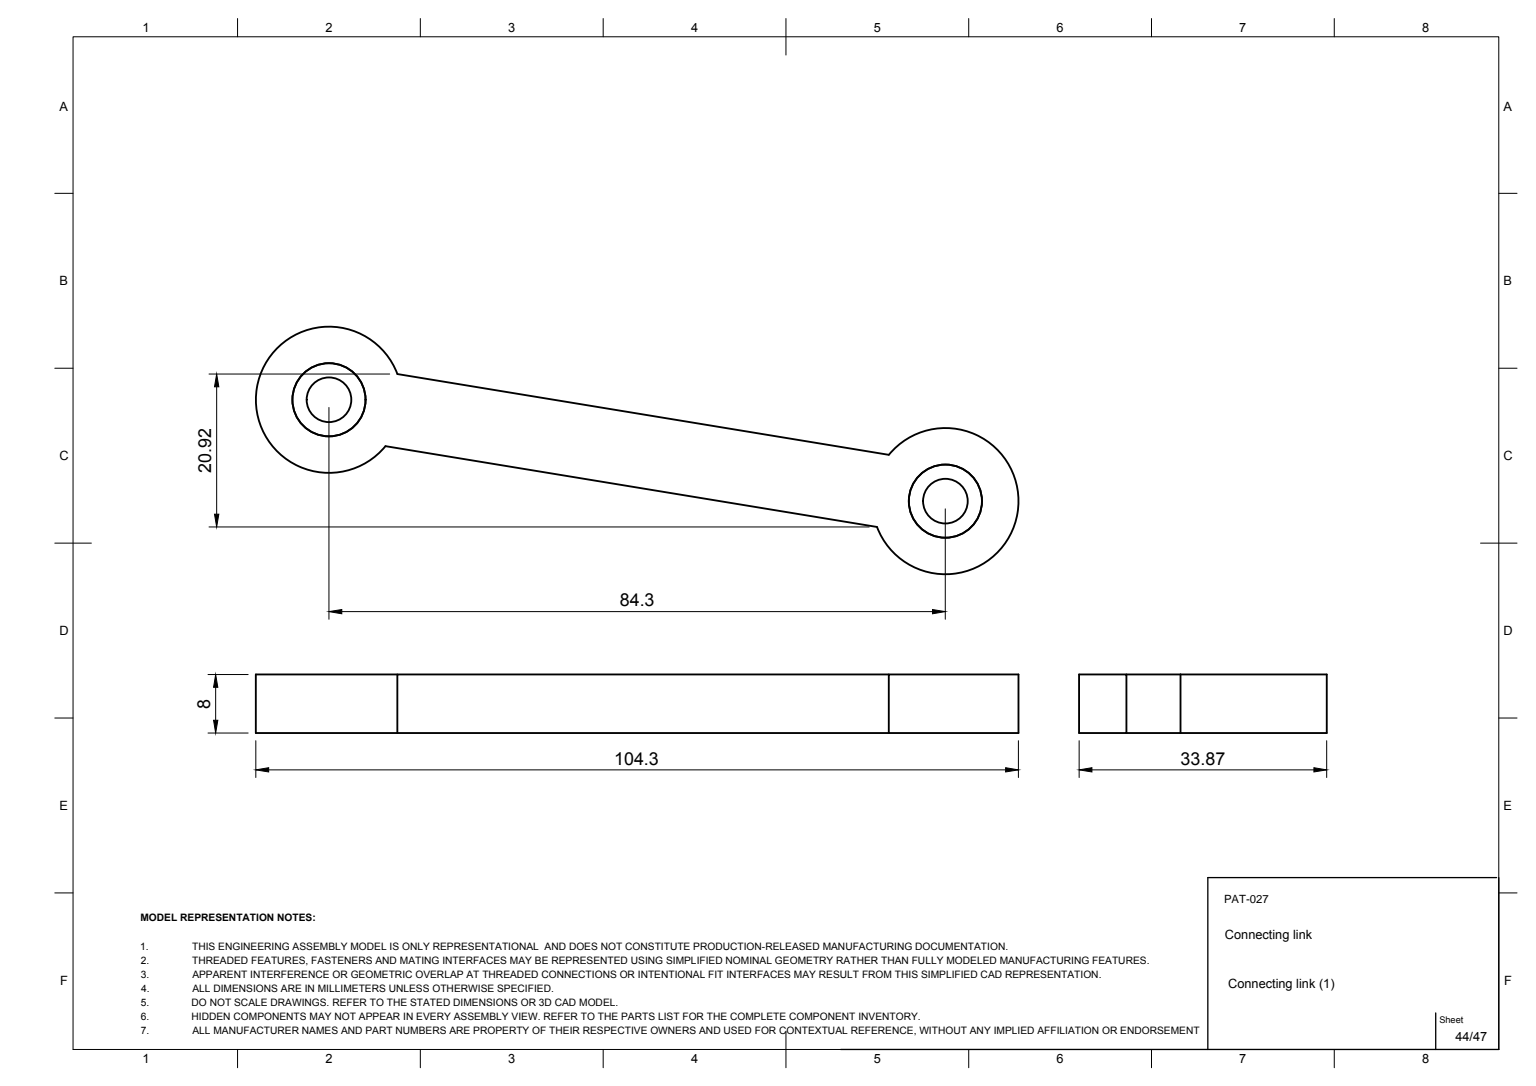
ISO-10303-21;
HEADER;
/* Generated by software containing ST-Developer
 * from STEP Tools, Inc. (www.steptools.com) 
 */

FILE_DESCRIPTION(
/* description */ ('Crank-driven oscillating fan base (mechanism only)'),

/* implementation_level */ '2;1');

FILE_NAME(
/* name */ 'Connecting link.step',
/* time_stamp */ '2026-10-28T03:25:00-07:00',
/* author */ (''),
/* organization */ (''),
/* preprocessor_version */ 'ST-DEVELOPER v20.2',
/* originating_system */ 'Autodesk Translation Framework v15.17.0.0',
/* authorisation */ '');

FILE_SCHEMA (('AUTOMOTIVE_DESIGN { 1 0 10303 214 3 1 1 }'));
ENDSEC;

DATA;
#10=MECHANICAL_DESIGN_GEOMETRIC_PRESENTATION_REPRESENTATION('',(#482),#11916);
#394=SHAPE_REPRESENTATION_RELATIONSHIP('SRR','None',#12122,#434);
#434=ADVANCED_BREP_SHAPE_REPRESENTATION('',(#527),#11913);
#482=STYLED_ITEM('',(#12368),#527);
#527=MANIFOLD_SOLID_BREP('Body1',#6115);
#684=FACE_BOUND('',#1779,.T.);
#685=FACE_BOUND('',#1780,.T.);
#686=FACE_BOUND('',#1784,.T.);
#687=FACE_BOUND('',#1785,.T.);
#878=PLANE('',#7379);
#879=PLANE('',#7380);
#880=PLANE('',#7382);
#881=PLANE('',#7385);
#1245=FACE_OUTER_BOUND('',#1774,.T.);
#1246=FACE_OUTER_BOUND('',#1775,.T.);
#1247=FACE_OUTER_BOUND('',#1776,.T.);
#1248=FACE_OUTER_BOUND('',#1777,.T.);
#1249=FACE_OUTER_BOUND('',#1778,.T.);
#1250=FACE_OUTER_BOUND('',#1781,.T.);
#1251=FACE_OUTER_BOUND('',#1782,.T.);
#1252=FACE_OUTER_BOUND('',#1783,.T.);
#1774=EDGE_LOOP('',(#5486,#5487,#5488,#5489));
#1775=EDGE_LOOP('',(#5490,#5491,#5492,#5493));
#1776=EDGE_LOOP('',(#5494,#5495,#5496,#5497));
#1777=EDGE_LOOP('',(#5498,#5499,#5500,#5501));
#1778=EDGE_LOOP('',(#5502,#5503,#5504,#5505));
#1779=EDGE_LOOP('',(#5506));
#1780=EDGE_LOOP('',(#5507));
#1781=EDGE_LOOP('',(#5508,#5509,#5510,#5511));
#1782=EDGE_LOOP('',(#5512,#5513,#5514,#5515));
#1783=EDGE_LOOP('',(#5516,#5517,#5518,#5519));
#1784=EDGE_LOOP('',(#5520));
#1785=EDGE_LOOP('',(#5521));
#2117=LINE('',#11752,#2450);
#2118=LINE('',#11758,#2451);
#2119=LINE('',#11763,#2452);
#2120=LINE('',#11767,#2453);
#2121=LINE('',#11771,#2454);
#2122=LINE('',#11773,#2455);
#2123=LINE('',#11774,#2456);
#2124=LINE('',#11777,#2457);
#2125=LINE('',#11781,#2458);
#2126=LINE('',#11782,#2459);
#2450=VECTOR('',#9356,0.5);
#2451=VECTOR('',#9363,0.5);
#2452=VECTOR('',#9368,1.);
#2453=VECTOR('',#9371,1.);
#2454=VECTOR('',#9376,1.);
#2455=VECTOR('',#9377,1.);
#2456=VECTOR('',#9378,1.);
#2457=VECTOR('',#9381,1.);
#2458=VECTOR('',#9386,1.);
#2459=VECTOR('',#9387,1.);
#2813=CIRCLE('',#7371,0.5);
#2814=CIRCLE('',#7372,0.5);
#2815=CIRCLE('',#7374,0.5);
#2816=CIRCLE('',#7375,0.5);
#2817=CIRCLE('',#7377,1.);
#2818=CIRCLE('',#7378,1.);
#2819=CIRCLE('',#7381,1.);
#2820=CIRCLE('',#7384,1.);
#3309=VERTEX_POINT('',#11749);
#3310=VERTEX_POINT('',#11751);
#3311=VERTEX_POINT('',#11755);
#3312=VERTEX_POINT('',#11757);
#3313=VERTEX_POINT('',#11761);
#3314=VERTEX_POINT('',#11762);
#3315=VERTEX_POINT('',#11764);
#3316=VERTEX_POINT('',#11766);
#3317=VERTEX_POINT('',#11770);
#3318=VERTEX_POINT('',#11772);
#3319=VERTEX_POINT('',#11776);
#3320=VERTEX_POINT('',#11780);
#4038=EDGE_CURVE('',#3309,#3309,#2813,.T.);
#4039=EDGE_CURVE('',#3309,#3310,#2117,.T.);
#4040=EDGE_CURVE('',#3310,#3310,#2814,.T.);
#4041=EDGE_CURVE('',#3311,#3311,#2815,.T.);
#4042=EDGE_CURVE('',#3311,#3312,#2118,.T.);
#4043=EDGE_CURVE('',#3312,#3312,#2816,.T.);
#4044=EDGE_CURVE('',#3313,#3314,#2119,.T.);
#4045=EDGE_CURVE('',#3315,#3313,#2817,.T.);
#4046=EDGE_CURVE('',#3316,#3315,#2120,.T.);
#4047=EDGE_CURVE('',#3316,#3314,#2818,.T.);
#4048=EDGE_CURVE('',#3317,#3314,#2121,.T.);
#4049=EDGE_CURVE('',#3318,#3317,#2122,.T.);
#4050=EDGE_CURVE('',#3313,#3318,#2123,.T.);
#4051=EDGE_CURVE('',#3316,#3319,#2124,.T.);
#4052=EDGE_CURVE('',#3317,#3319,#2819,.T.);
#4053=EDGE_CURVE('',#3320,#3315,#2125,.T.);
#4054=EDGE_CURVE('',#3319,#3320,#2126,.T.);
#4055=EDGE_CURVE('',#3318,#3320,#2820,.T.);
#5486=ORIENTED_EDGE('',*,*,#4038,.F.);
#5487=ORIENTED_EDGE('',*,*,#4039,.T.);
#5488=ORIENTED_EDGE('',*,*,#4040,.F.);
#5489=ORIENTED_EDGE('',*,*,#4039,.F.);
#5490=ORIENTED_EDGE('',*,*,#4041,.F.);
#5491=ORIENTED_EDGE('',*,*,#4042,.T.);
#5492=ORIENTED_EDGE('',*,*,#4043,.F.);
#5493=ORIENTED_EDGE('',*,*,#4042,.F.);
#5494=ORIENTED_EDGE('',*,*,#4044,.F.);
#5495=ORIENTED_EDGE('',*,*,#4045,.F.);
#5496=ORIENTED_EDGE('',*,*,#4046,.F.);
#5497=ORIENTED_EDGE('',*,*,#4047,.T.);
#5498=ORIENTED_EDGE('',*,*,#4044,.T.);
#5499=ORIENTED_EDGE('',*,*,#4048,.F.);
#5500=ORIENTED_EDGE('',*,*,#4049,.F.);
#5501=ORIENTED_EDGE('',*,*,#4050,.F.);
#5502=ORIENTED_EDGE('',*,*,#4047,.F.);
#5503=ORIENTED_EDGE('',*,*,#4051,.T.);
#5504=ORIENTED_EDGE('',*,*,#4052,.F.);
#5505=ORIENTED_EDGE('',*,*,#4048,.T.);
#5506=ORIENTED_EDGE('',*,*,#4038,.T.);
#5507=ORIENTED_EDGE('',*,*,#4041,.T.);
#5508=ORIENTED_EDGE('',*,*,#4046,.T.);
#5509=ORIENTED_EDGE('',*,*,#4053,.F.);
#5510=ORIENTED_EDGE('',*,*,#4054,.F.);
#5511=ORIENTED_EDGE('',*,*,#4051,.F.);
#5512=ORIENTED_EDGE('',*,*,#4049,.T.);
#5513=ORIENTED_EDGE('',*,*,#4052,.T.);
#5514=ORIENTED_EDGE('',*,*,#4054,.T.);
#5515=ORIENTED_EDGE('',*,*,#4055,.F.);
#5516=ORIENTED_EDGE('',*,*,#4050,.T.);
#5517=ORIENTED_EDGE('',*,*,#4055,.T.);
#5518=ORIENTED_EDGE('',*,*,#4053,.T.);
#5519=ORIENTED_EDGE('',*,*,#4045,.T.);
#5520=ORIENTED_EDGE('',*,*,#4040,.T.);
#5521=ORIENTED_EDGE('',*,*,#4043,.T.);
#5684=CYLINDRICAL_SURFACE('',#7370,0.5);
#5685=CYLINDRICAL_SURFACE('',#7373,0.5);
#5686=CYLINDRICAL_SURFACE('',#7376,1.);
#5687=CYLINDRICAL_SURFACE('',#7383,1.);
#6051=ADVANCED_FACE('',(#1245),#5684,.F.);
#6052=ADVANCED_FACE('',(#1246),#5685,.F.);
#6053=ADVANCED_FACE('',(#1247),#5686,.T.);
#6054=ADVANCED_FACE('',(#1248),#878,.T.);
#6055=ADVANCED_FACE('',(#1249,#684,#685),#879,.F.);
#6056=ADVANCED_FACE('',(#1250),#880,.T.);
#6057=ADVANCED_FACE('',(#1251),#5687,.T.);
#6058=ADVANCED_FACE('',(#1252,#686,#687),#881,.T.);
#6115=CLOSED_SHELL('',(#6051,#6052,#6053,#6054,#6055,#6056,#6057,#6058));
#7369=AXIS2_PLACEMENT_3D('',#11747,#9350,#9351);
#7370=AXIS2_PLACEMENT_3D('',#11748,#9352,#9353);
#7371=AXIS2_PLACEMENT_3D('',#11750,#9354,#9355);
#7372=AXIS2_PLACEMENT_3D('',#11753,#9357,#9358);
#7373=AXIS2_PLACEMENT_3D('',#11754,#9359,#9360);
#7374=AXIS2_PLACEMENT_3D('',#11756,#9361,#9362);
#7375=AXIS2_PLACEMENT_3D('',#11759,#9364,#9365);
#7376=AXIS2_PLACEMENT_3D('',#11760,#9366,#9367);
#7377=AXIS2_PLACEMENT_3D('',#11765,#9369,#9370);
#7378=AXIS2_PLACEMENT_3D('',#11768,#9372,#9373);
#7379=AXIS2_PLACEMENT_3D('',#11769,#9374,#9375);
#7380=AXIS2_PLACEMENT_3D('',#11775,#9379,#9380);
#7381=AXIS2_PLACEMENT_3D('',#11778,#9382,#9383);
#7382=AXIS2_PLACEMENT_3D('',#11779,#9384,#9385);
#7383=AXIS2_PLACEMENT_3D('',#11783,#9388,#9389);
#7384=AXIS2_PLACEMENT_3D('',#11784,#9390,#9391);
#7385=AXIS2_PLACEMENT_3D('',#11785,#9392,#9393);
#9350=DIRECTION('axis',(0.,0.,1.));
#9351=DIRECTION('refdir',(1.,0.,0.));
#9352=DIRECTION('center_axis',(0.,0.,1.));
#9353=DIRECTION('ref_axis',(1.,0.,0.));
#9354=DIRECTION('center_axis',(0.,0.,1.));
#9355=DIRECTION('ref_axis',(1.,0.,0.));
#9356=DIRECTION('',(0.,0.,1.));
#9357=DIRECTION('center_axis',(0.,0.,-1.));
#9358=DIRECTION('ref_axis',(1.,0.,0.));
#9359=DIRECTION('center_axis',(0.,0.,1.));
#9360=DIRECTION('ref_axis',(1.,0.,0.));
#9361=DIRECTION('center_axis',(0.,0.,1.));
#9362=DIRECTION('ref_axis',(1.,0.,0.));
#9363=DIRECTION('',(0.,0.,1.));
#9364=DIRECTION('center_axis',(0.,0.,-1.));
#9365=DIRECTION('ref_axis',(1.,0.,0.));
#9366=DIRECTION('center_axis',(0.,0.,1.));
#9367=DIRECTION('ref_axis',(1.,0.,0.));
#9368=DIRECTION('',(0.,0.,-1.));
#9369=DIRECTION('center_axis',(0.,0.,1.));
#9370=DIRECTION('ref_axis',(1.,0.,0.));
#9371=DIRECTION('',(0.,0.,1.));
#9372=DIRECTION('center_axis',(0.,0.,1.));
#9373=DIRECTION('ref_axis',(1.,0.,0.));
#9374=DIRECTION('center_axis',(-0.162294462269189,0.986742371400334,0.));
#9375=DIRECTION('ref_axis',(-0.986742371400334,-0.162294462269189,0.));
#9376=DIRECTION('',(0.986742371400334,0.162294462269189,0.));
#9377=DIRECTION('',(0.,0.,-1.));
#9378=DIRECTION('',(-0.986742371400334,-0.162294462269189,0.));
#9379=DIRECTION('center_axis',(0.,0.,1.));
#9380=DIRECTION('ref_axis',(1.,0.,0.));
#9381=DIRECTION('',(-0.986742371400334,-0.162294462269189,0.));
#9382=DIRECTION('center_axis',(0.,0.,1.));
#9383=DIRECTION('ref_axis',(1.,0.,0.));
#9384=DIRECTION('center_axis',(0.162294462269189,-0.986742371400334,0.));
#9385=DIRECTION('ref_axis',(0.986742371400334,0.162294462269189,0.));
#9386=DIRECTION('',(0.986742371400334,0.162294462269189,0.));
#9387=DIRECTION('',(0.,0.,1.));
#9388=DIRECTION('center_axis',(0.,0.,1.));
#9389=DIRECTION('ref_axis',(-0.986742371400334,-0.162294462269189,0.));
#9390=DIRECTION('center_axis',(0.,0.,1.));
#9391=DIRECTION('ref_axis',(1.,0.,0.));
#9392=DIRECTION('center_axis',(0.,0.,1.));
#9393=DIRECTION('ref_axis',(1.,0.,0.));
#11747=CARTESIAN_POINT('',(0.,0.,0.));
#11748=CARTESIAN_POINT('Origin',(-0.429855350392604,2.61349944954989,8.5));
#11749=CARTESIAN_POINT('',(-0.929855350392604,2.61349944954989,8.6));
#11750=CARTESIAN_POINT('Origin',(-0.429855350392604,2.61349944954989,8.6));
#11751=CARTESIAN_POINT('',(-0.929855350392604,2.61349944954989,9.4));
#11752=CARTESIAN_POINT('',(-0.929855350392604,2.61349944954989,8.5));
#11753=CARTESIAN_POINT('Origin',(-0.429855350392604,2.61349944954989,9.4));
#11754=CARTESIAN_POINT('Origin',(8.,4.,8.5));
#11755=CARTESIAN_POINT('',(7.5,4.,8.6));
#11756=CARTESIAN_POINT('Origin',(8.,4.,8.6));
#11757=CARTESIAN_POINT('',(7.5,4.,9.4));
#11758=CARTESIAN_POINT('',(7.5,4.,8.5));
#11759=CARTESIAN_POINT('Origin',(8.,4.,9.4));
#11760=CARTESIAN_POINT('Origin',(8.,4.,8.6));
#11761=CARTESIAN_POINT('',(7.06430880824222,4.35282005848151,9.4));
#11762=CARTESIAN_POINT('',(7.06430880824222,4.35282005848151,8.6));
#11763=CARTESIAN_POINT('',(7.06430880824222,4.35282005848151,8.6));
#11764=CARTESIAN_POINT('',(7.22660327051141,3.36607768708118,9.4));
#11765=CARTESIAN_POINT('Origin',(8.,4.,9.4));
#11766=CARTESIAN_POINT('',(7.22660327051141,3.36607768708118,8.6));
#11767=CARTESIAN_POINT('',(7.22660327051141,3.36607768708118,8.6));
#11768=CARTESIAN_POINT('Origin',(8.,4.,8.6));
#11769=CARTESIAN_POINT('Origin',(7.91885276886541,4.49337118570017,8.6));
#11770=CARTESIAN_POINT('',(0.34354137909599,3.24742176246871,8.6));
#11771=CARTESIAN_POINT('',(-0.511002581527199,3.10687063525006,8.6));
#11772=CARTESIAN_POINT('',(0.34354137909599,3.24742176246871,9.4));
#11773=CARTESIAN_POINT('',(0.343541379095991,3.24742176246871,8.6));
#11774=CARTESIAN_POINT('',(-0.511002581527199,3.10687063525006,9.4));
#11775=CARTESIAN_POINT('Origin',(-0.429855350392604,2.61349944954989,8.6));
#11776=CARTESIAN_POINT('',(0.505835841365177,2.26067939106837,8.6));
#11777=CARTESIAN_POINT('',(8.08114723113459,3.50662881429983,8.6));
#11778=CARTESIAN_POINT('Origin',(-0.429855350392604,2.61349944954989,8.6));
#11779=CARTESIAN_POINT('Origin',(-0.34870811925801,2.12012826384972,8.6));
#11780=CARTESIAN_POINT('',(0.505835841365177,2.26067939106837,9.4));
#11781=CARTESIAN_POINT('',(8.08114723113459,3.50662881429983,9.4));
#11782=CARTESIAN_POINT('',(0.505835841365179,2.26067939106837,8.6));
#11783=CARTESIAN_POINT('Origin',(-0.429855350392604,2.61349944954989,8.6));
#11784=CARTESIAN_POINT('Origin',(-0.429855350392604,2.61349944954989,9.4));
#11785=CARTESIAN_POINT('Origin',(-0.429855350392604,2.61349944954989,9.4));
#11866=UNCERTAINTY_MEASURE_WITH_UNIT(LENGTH_MEASURE(0.001),#11917,
'DISTANCE_ACCURACY_VALUE',
'Maximum model space distance between geometric entities at asserted c
onnectivities');
#11869=UNCERTAINTY_MEASURE_WITH_UNIT(LENGTH_MEASURE(0.001),#11917,
'DISTANCE_ACCURACY_VALUE',
'Maximum model space distance between geometric entities at asserted c
onnectivities');
#11913=(
GEOMETRIC_REPRESENTATION_CONTEXT(3)
GLOBAL_UNCERTAINTY_ASSIGNED_CONTEXT((#11866))
GLOBAL_UNIT_ASSIGNED_CONTEXT((#11917,#11919,#11920))
REPRESENTATION_CONTEXT('','3D')
);
#11916=(
GEOMETRIC_REPRESENTATION_CONTEXT(3)
GLOBAL_UNCERTAINTY_ASSIGNED_CONTEXT((#11869))
GLOBAL_UNIT_ASSIGNED_CONTEXT((#11917,#11919,#11920))
REPRESENTATION_CONTEXT('','3D')
);
#11917=(
LENGTH_UNIT()
NAMED_UNIT(*)
SI_UNIT(.CENTI.,.METRE.)
);
#11919=(
NAMED_UNIT(*)
PLANE_ANGLE_UNIT()
SI_UNIT($,.RADIAN.)
);
#11920=(
NAMED_UNIT(*)
SI_UNIT($,.STERADIAN.)
SOLID_ANGLE_UNIT()
);
#11964=SHAPE_DEFINITION_REPRESENTATION(#12069,#12122);
#12069=PRODUCT_DEFINITION_SHAPE('',$,#12169);
#12122=SHAPE_REPRESENTATION('',(#7369),#11913);
#12125=PRODUCT_DEFINITION_CONTEXT('part definition',#12265,'design');
#12169=PRODUCT_DEFINITION('Connecting link','Connecting link',#12215,
#12125);
#12215=PRODUCT_DEFINITION_FORMATION('',$,#12310);
#12265=APPLICATION_CONTEXT(
'Core Data for Automotive Mechanical Design Process');
#12266=PRODUCT_CONTEXT('part definition',#12265,'mechanical');
#12310=PRODUCT('Connecting link','Connecting link','Connecting link',
(#12266));
#12362=COLOUR_RGB('Sky Blue',0.24,0.69,0.87);
#12363=FILL_AREA_STYLE_COLOUR('',#12362);
#12364=FILL_AREA_STYLE('',(#12363));
#12365=SURFACE_STYLE_FILL_AREA(#12364);
#12366=SURFACE_SIDE_STYLE('',(#12365));
#12367=SURFACE_STYLE_USAGE(.BOTH.,#12366);
#12368=PRESENTATION_STYLE_ASSIGNMENT((#12367));
ENDSEC;
END-ISO-10303-21;
